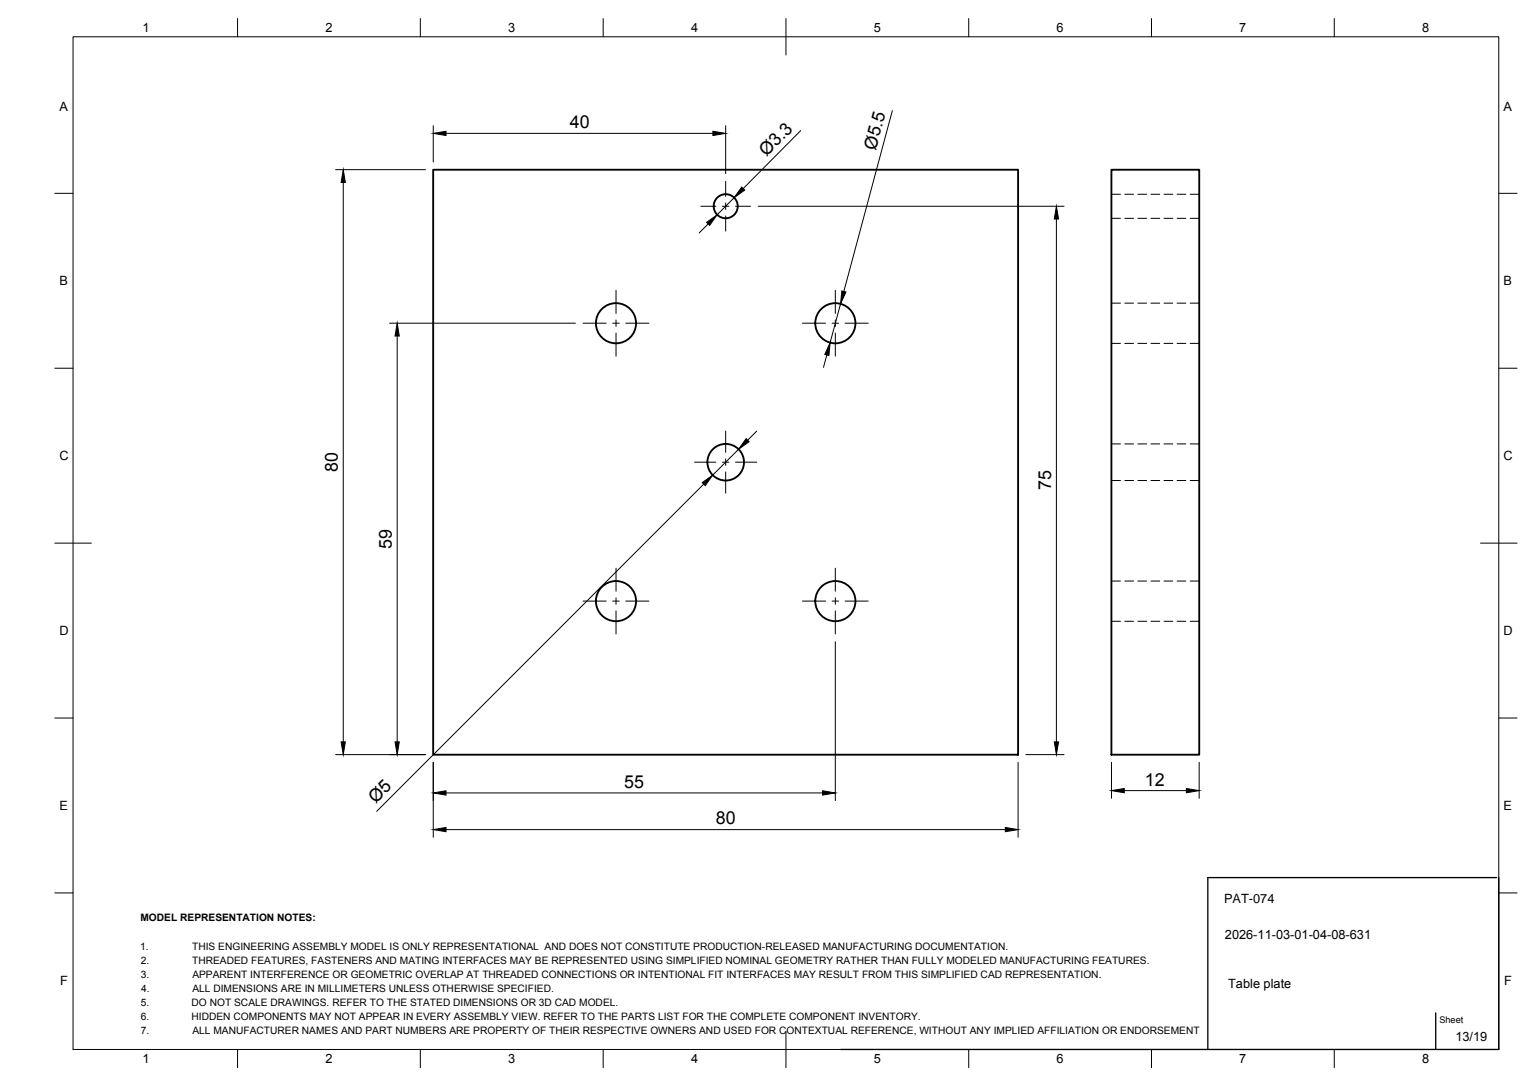
ISO-10303-21;
HEADER;
/* Generated by software containing ST-Developer
 * from STEP Tools, Inc. (www.steptools.com) 
 */

FILE_DESCRIPTION(
/* description */ ('Manual rail carriage with stops'),
/* implementation_level */ '2;1');

FILE_NAME(
/* name */ 'Table plate.step',
/* time_stamp */ '2026-10-27T18:54:27-07:00',
/* author */ (''),
/* organization */ (''),
/* preprocessor_version */ 'ST-DEVELOPER v20.2',
/* originating_system */ 'Autodesk Translation Framework v15.17.0.0',
/* authorisation */ '');

FILE_SCHEMA (('AUTOMOTIVE_DESIGN { 1 0 10303 214 3 1 1 }'));
ENDSEC;

DATA;
#10=MECHANICAL_DESIGN_GEOMETRIC_PRESENTATION_REPRESENTATION('',(#285),#8499);
#249=SHAPE_REPRESENTATION_RELATIONSHIP('SRR','None',#8614,#267);
#267=ADVANCED_BREP_SHAPE_REPRESENTATION('',(#301),#8493);
#285=STYLED_ITEM('',(#8781),#301);
#301=MANIFOLD_SOLID_BREP('Body1',#4955);
#360=FACE_BOUND('',#1114,.T.);
#361=FACE_BOUND('',#1115,.T.);
#362=FACE_BOUND('',#1116,.T.);
#363=FACE_BOUND('',#1117,.T.);
#364=FACE_BOUND('',#1118,.T.);
#365=FACE_BOUND('',#1119,.T.);
#366=FACE_BOUND('',#1121,.T.);
#367=FACE_BOUND('',#1122,.T.);
#368=FACE_BOUND('',#1123,.T.);
#369=FACE_BOUND('',#1124,.T.);
#370=FACE_BOUND('',#1125,.T.);
#371=FACE_BOUND('',#1126,.T.);
#543=PLANE('',#5497);
#544=PLANE('',#5498);
#545=PLANE('',#5499);
#546=PLANE('',#5500);
#547=PLANE('',#5501);
#548=PLANE('',#5502);
#783=FACE_OUTER_BOUND('',#1103,.T.);
#784=FACE_OUTER_BOUND('',#1104,.T.);
#785=FACE_OUTER_BOUND('',#1105,.T.);
#786=FACE_OUTER_BOUND('',#1106,.T.);
#787=FACE_OUTER_BOUND('',#1107,.T.);
#788=FACE_OUTER_BOUND('',#1108,.T.);
#789=FACE_OUTER_BOUND('',#1109,.T.);
#790=FACE_OUTER_BOUND('',#1110,.T.);
#791=FACE_OUTER_BOUND('',#1111,.T.);
#792=FACE_OUTER_BOUND('',#1112,.T.);
#793=FACE_OUTER_BOUND('',#1113,.T.);
#794=FACE_OUTER_BOUND('',#1120,.T.);
#1103=EDGE_LOOP('',(#4396,#4397,#4398,#4399));
#1104=EDGE_LOOP('',(#4400,#4401,#4402,#4403));
#1105=EDGE_LOOP('',(#4404,#4405,#4406,#4407));
#1106=EDGE_LOOP('',(#4408,#4409,#4410,#4411));
#1107=EDGE_LOOP('',(#4412,#4413,#4414,#4415));
#1108=EDGE_LOOP('',(#4416,#4417,#4418,#4419));
#1109=EDGE_LOOP('',(#4420,#4421,#4422,#4423));
#1110=EDGE_LOOP('',(#4424,#4425,#4426,#4427));
#1111=EDGE_LOOP('',(#4428,#4429,#4430,#4431));
#1112=EDGE_LOOP('',(#4432,#4433,#4434,#4435));
#1113=EDGE_LOOP('',(#4436,#4437,#4438,#4439));
#1114=EDGE_LOOP('',(#4440));
#1115=EDGE_LOOP('',(#4441));
#1116=EDGE_LOOP('',(#4442));
#1117=EDGE_LOOP('',(#4443));
#1118=EDGE_LOOP('',(#4444));
#1119=EDGE_LOOP('',(#4445));
#1120=EDGE_LOOP('',(#4446,#4447,#4448,#4449));
#1121=EDGE_LOOP('',(#4450));
#1122=EDGE_LOOP('',(#4451));
#1123=EDGE_LOOP('',(#4452));
#1124=EDGE_LOOP('',(#4453));
#1125=EDGE_LOOP('',(#4454));
#1126=EDGE_LOOP('',(#4455));
#1609=LINE('',#8160,#2109);
#1610=LINE('',#8166,#2110);
#1611=LINE('',#8172,#2111);
#1612=LINE('',#8178,#2112);
#1613=LINE('',#8184,#2113);
#1614=LINE('',#8190,#2114);
#1615=LINE('',#8195,#2115);
#1616=LINE('',#8197,#2116);
#1617=LINE('',#8199,#2117);
#1618=LINE('',#8200,#2118);
#1619=LINE('',#8203,#2119);
#1620=LINE('',#8205,#2120);
#1621=LINE('',#8206,#2121);
#1622=LINE('',#8209,#2122);
#1623=LINE('',#8211,#2123);
#1624=LINE('',#8212,#2124);
#1625=LINE('',#8214,#2125);
#1626=LINE('',#8215,#2126);
#2109=VECTOR('',#6696,0.164999999999999);
#2110=VECTOR('',#6703,0.25);
#2111=VECTOR('',#6710,0.275);
#2112=VECTOR('',#6717,0.275);
#2113=VECTOR('',#6724,0.275);
#2114=VECTOR('',#6731,0.275);
#2115=VECTOR('',#6736,1.);
#2116=VECTOR('',#6737,1.);
#2117=VECTOR('',#6738,1.);
#2118=VECTOR('',#6739,1.);
#2119=VECTOR('',#6742,1.);
#2120=VECTOR('',#6743,1.);
#2121=VECTOR('',#6744,1.);
#2122=VECTOR('',#6747,1.);
#2123=VECTOR('',#6748,1.);
#2124=VECTOR('',#6749,1.);
#2125=VECTOR('',#6752,1.);
#2126=VECTOR('',#6753,1.);
#2271=CIRCLE('',#5480,0.164999999999999);
#2272=CIRCLE('',#5481,0.164999999999999);
#2273=CIRCLE('',#5483,0.25);
#2274=CIRCLE('',#5484,0.25);
#2275=CIRCLE('',#5486,0.275);
#2276=CIRCLE('',#5487,0.275);
#2277=CIRCLE('',#5489,0.275);
#2278=CIRCLE('',#5490,0.275);
#2279=CIRCLE('',#5492,0.275);
#2280=CIRCLE('',#5493,0.275);
#2281=CIRCLE('',#5495,0.275);
#2282=CIRCLE('',#5496,0.275);
#2655=VERTEX_POINT('',#8157);
#2656=VERTEX_POINT('',#8159);
#2657=VERTEX_POINT('',#8163);
#2658=VERTEX_POINT('',#8165);
#2659=VERTEX_POINT('',#8169);
#2660=VERTEX_POINT('',#8171);
#2661=VERTEX_POINT('',#8175);
#2662=VERTEX_POINT('',#8177);
#2663=VERTEX_POINT('',#8181);
#2664=VERTEX_POINT('',#8183);
#2665=VERTEX_POINT('',#8187);
#2666=VERTEX_POINT('',#8189);
#2667=VERTEX_POINT('',#8193);
#2668=VERTEX_POINT('',#8194);
#2669=VERTEX_POINT('',#8196);
#2670=VERTEX_POINT('',#8198);
#2671=VERTEX_POINT('',#8202);
#2672=VERTEX_POINT('',#8204);
#2673=VERTEX_POINT('',#8208);
#2674=VERTEX_POINT('',#8210);
#3246=EDGE_CURVE('',#2655,#2655,#2271,.T.);
#3247=EDGE_CURVE('',#2655,#2656,#1609,.T.);
#3248=EDGE_CURVE('',#2656,#2656,#2272,.T.);
#3249=EDGE_CURVE('',#2657,#2657,#2273,.T.);
#3250=EDGE_CURVE('',#2657,#2658,#1610,.T.);
#3251=EDGE_CURVE('',#2658,#2658,#2274,.T.);
#3252=EDGE_CURVE('',#2659,#2659,#2275,.T.);
#3253=EDGE_CURVE('',#2659,#2660,#1611,.T.);
#3254=EDGE_CURVE('',#2660,#2660,#2276,.T.);
#3255=EDGE_CURVE('',#2661,#2661,#2277,.T.);
#3256=EDGE_CURVE('',#2661,#2662,#1612,.T.);
#3257=EDGE_CURVE('',#2662,#2662,#2278,.T.);
#3258=EDGE_CURVE('',#2663,#2663,#2279,.T.);
#3259=EDGE_CURVE('',#2663,#2664,#1613,.T.);
#3260=EDGE_CURVE('',#2664,#2664,#2280,.T.);
#3261=EDGE_CURVE('',#2665,#2665,#2281,.T.);
#3262=EDGE_CURVE('',#2665,#2666,#1614,.T.);
#3263=EDGE_CURVE('',#2666,#2666,#2282,.T.);
#3264=EDGE_CURVE('',#2667,#2668,#1615,.T.);
#3265=EDGE_CURVE('',#2668,#2669,#1616,.T.);
#3266=EDGE_CURVE('',#2670,#2669,#1617,.T.);
#3267=EDGE_CURVE('',#2667,#2670,#1618,.T.);
#3268=EDGE_CURVE('',#2671,#2667,#1619,.T.);
#3269=EDGE_CURVE('',#2672,#2670,#1620,.T.);
#3270=EDGE_CURVE('',#2671,#2672,#1621,.T.);
#3271=EDGE_CURVE('',#2673,#2671,#1622,.T.);
#3272=EDGE_CURVE('',#2674,#2672,#1623,.T.);
#3273=EDGE_CURVE('',#2673,#2674,#1624,.T.);
#3274=EDGE_CURVE('',#2668,#2673,#1625,.T.);
#3275=EDGE_CURVE('',#2669,#2674,#1626,.T.);
#4396=ORIENTED_EDGE('',*,*,#3246,.F.);
#4397=ORIENTED_EDGE('',*,*,#3247,.T.);
#4398=ORIENTED_EDGE('',*,*,#3248,.F.);
#4399=ORIENTED_EDGE('',*,*,#3247,.F.);
#4400=ORIENTED_EDGE('',*,*,#3249,.F.);
#4401=ORIENTED_EDGE('',*,*,#3250,.T.);
#4402=ORIENTED_EDGE('',*,*,#3251,.F.);
#4403=ORIENTED_EDGE('',*,*,#3250,.F.);
#4404=ORIENTED_EDGE('',*,*,#3252,.F.);
#4405=ORIENTED_EDGE('',*,*,#3253,.T.);
#4406=ORIENTED_EDGE('',*,*,#3254,.F.);
#4407=ORIENTED_EDGE('',*,*,#3253,.F.);
#4408=ORIENTED_EDGE('',*,*,#3255,.F.);
#4409=ORIENTED_EDGE('',*,*,#3256,.T.);
#4410=ORIENTED_EDGE('',*,*,#3257,.F.);
#4411=ORIENTED_EDGE('',*,*,#3256,.F.);
#4412=ORIENTED_EDGE('',*,*,#3258,.F.);
#4413=ORIENTED_EDGE('',*,*,#3259,.T.);
#4414=ORIENTED_EDGE('',*,*,#3260,.F.);
#4415=ORIENTED_EDGE('',*,*,#3259,.F.);
#4416=ORIENTED_EDGE('',*,*,#3261,.F.);
#4417=ORIENTED_EDGE('',*,*,#3262,.T.);
#4418=ORIENTED_EDGE('',*,*,#3263,.F.);
#4419=ORIENTED_EDGE('',*,*,#3262,.F.);
#4420=ORIENTED_EDGE('',*,*,#3264,.T.);
#4421=ORIENTED_EDGE('',*,*,#3265,.T.);
#4422=ORIENTED_EDGE('',*,*,#3266,.F.);
#4423=ORIENTED_EDGE('',*,*,#3267,.F.);
#4424=ORIENTED_EDGE('',*,*,#3268,.T.);
#4425=ORIENTED_EDGE('',*,*,#3267,.T.);
#4426=ORIENTED_EDGE('',*,*,#3269,.F.);
#4427=ORIENTED_EDGE('',*,*,#3270,.F.);
#4428=ORIENTED_EDGE('',*,*,#3271,.T.);
#4429=ORIENTED_EDGE('',*,*,#3270,.T.);
#4430=ORIENTED_EDGE('',*,*,#3272,.F.);
#4431=ORIENTED_EDGE('',*,*,#3273,.F.);
#4432=ORIENTED_EDGE('',*,*,#3274,.T.);
#4433=ORIENTED_EDGE('',*,*,#3273,.T.);
#4434=ORIENTED_EDGE('',*,*,#3275,.F.);
#4435=ORIENTED_EDGE('',*,*,#3265,.F.);
#4436=ORIENTED_EDGE('',*,*,#3275,.T.);
#4437=ORIENTED_EDGE('',*,*,#3272,.T.);
#4438=ORIENTED_EDGE('',*,*,#3269,.T.);
#4439=ORIENTED_EDGE('',*,*,#3266,.T.);
#4440=ORIENTED_EDGE('',*,*,#3248,.T.);
#4441=ORIENTED_EDGE('',*,*,#3251,.T.);
#4442=ORIENTED_EDGE('',*,*,#3254,.T.);
#4443=ORIENTED_EDGE('',*,*,#3257,.T.);
#4444=ORIENTED_EDGE('',*,*,#3260,.T.);
#4445=ORIENTED_EDGE('',*,*,#3263,.T.);
#4446=ORIENTED_EDGE('',*,*,#3274,.F.);
#4447=ORIENTED_EDGE('',*,*,#3264,.F.);
#4448=ORIENTED_EDGE('',*,*,#3268,.F.);
#4449=ORIENTED_EDGE('',*,*,#3271,.F.);
#4450=ORIENTED_EDGE('',*,*,#3246,.T.);
#4451=ORIENTED_EDGE('',*,*,#3249,.T.);
#4452=ORIENTED_EDGE('',*,*,#3252,.T.);
#4453=ORIENTED_EDGE('',*,*,#3255,.T.);
#4454=ORIENTED_EDGE('',*,*,#3258,.T.);
#4455=ORIENTED_EDGE('',*,*,#3261,.T.);
#4660=CYLINDRICAL_SURFACE('',#5479,0.164999999999999);
#4661=CYLINDRICAL_SURFACE('',#5482,0.25);
#4662=CYLINDRICAL_SURFACE('',#5485,0.275);
#4663=CYLINDRICAL_SURFACE('',#5488,0.275);
#4664=CYLINDRICAL_SURFACE('',#5491,0.275);
#4665=CYLINDRICAL_SURFACE('',#5494,0.275);
#4882=ADVANCED_FACE('',(#783),#4660,.F.);
#4883=ADVANCED_FACE('',(#784),#4661,.F.);
#4884=ADVANCED_FACE('',(#785),#4662,.F.);
#4885=ADVANCED_FACE('',(#786),#4663,.F.);
#4886=ADVANCED_FACE('',(#787),#4664,.F.);
#4887=ADVANCED_FACE('',(#788),#4665,.F.);
#4888=ADVANCED_FACE('',(#789),#543,.T.);
#4889=ADVANCED_FACE('',(#790),#544,.T.);
#4890=ADVANCED_FACE('',(#791),#545,.T.);
#4891=ADVANCED_FACE('',(#792),#546,.T.);
#4892=ADVANCED_FACE('',(#793,#360,#361,#362,#363,#364,#365),#547,.T.);
#4893=ADVANCED_FACE('',(#794,#366,#367,#368,#369,#370,#371),#548,.F.);
#4955=CLOSED_SHELL('',(#4882,#4883,#4884,#4885,#4886,#4887,#4888,#4889,
#4890,#4891,#4892,#4893));
#5478=AXIS2_PLACEMENT_3D('',#8155,#6690,#6691);
#5479=AXIS2_PLACEMENT_3D('',#8156,#6692,#6693);
#5480=AXIS2_PLACEMENT_3D('',#8158,#6694,#6695);
#5481=AXIS2_PLACEMENT_3D('',#8161,#6697,#6698);
#5482=AXIS2_PLACEMENT_3D('',#8162,#6699,#6700);
#5483=AXIS2_PLACEMENT_3D('',#8164,#6701,#6702);
#5484=AXIS2_PLACEMENT_3D('',#8167,#6704,#6705);
#5485=AXIS2_PLACEMENT_3D('',#8168,#6706,#6707);
#5486=AXIS2_PLACEMENT_3D('',#8170,#6708,#6709);
#5487=AXIS2_PLACEMENT_3D('',#8173,#6711,#6712);
#5488=AXIS2_PLACEMENT_3D('',#8174,#6713,#6714);
#5489=AXIS2_PLACEMENT_3D('',#8176,#6715,#6716);
#5490=AXIS2_PLACEMENT_3D('',#8179,#6718,#6719);
#5491=AXIS2_PLACEMENT_3D('',#8180,#6720,#6721);
#5492=AXIS2_PLACEMENT_3D('',#8182,#6722,#6723);
#5493=AXIS2_PLACEMENT_3D('',#8185,#6725,#6726);
#5494=AXIS2_PLACEMENT_3D('',#8186,#6727,#6728);
#5495=AXIS2_PLACEMENT_3D('',#8188,#6729,#6730);
#5496=AXIS2_PLACEMENT_3D('',#8191,#6732,#6733);
#5497=AXIS2_PLACEMENT_3D('',#8192,#6734,#6735);
#5498=AXIS2_PLACEMENT_3D('',#8201,#6740,#6741);
#5499=AXIS2_PLACEMENT_3D('',#8207,#6745,#6746);
#5500=AXIS2_PLACEMENT_3D('',#8213,#6750,#6751);
#5501=AXIS2_PLACEMENT_3D('',#8216,#6754,#6755);
#5502=AXIS2_PLACEMENT_3D('',#8217,#6756,#6757);
#6690=DIRECTION('axis',(0.,0.,1.));
#6691=DIRECTION('refdir',(1.,0.,0.));
#6692=DIRECTION('center_axis',(0.,0.,1.));
#6693=DIRECTION('ref_axis',(1.,0.,0.));
#6694=DIRECTION('center_axis',(0.,0.,1.));
#6695=DIRECTION('ref_axis',(1.,0.,0.));
#6696=DIRECTION('',(0.,0.,1.));
#6697=DIRECTION('center_axis',(0.,0.,-1.));
#6698=DIRECTION('ref_axis',(1.,0.,0.));
#6699=DIRECTION('center_axis',(0.,0.,1.));
#6700=DIRECTION('ref_axis',(1.,0.,0.));
#6701=DIRECTION('center_axis',(0.,0.,1.));
#6702=DIRECTION('ref_axis',(1.,0.,0.));
#6703=DIRECTION('',(0.,0.,1.));
#6704=DIRECTION('center_axis',(0.,0.,-1.));
#6705=DIRECTION('ref_axis',(1.,0.,0.));
#6706=DIRECTION('center_axis',(0.,0.,1.));
#6707=DIRECTION('ref_axis',(1.,0.,0.));
#6708=DIRECTION('center_axis',(0.,0.,1.));
#6709=DIRECTION('ref_axis',(1.,0.,0.));
#6710=DIRECTION('',(0.,0.,1.));
#6711=DIRECTION('center_axis',(0.,0.,-1.));
#6712=DIRECTION('ref_axis',(1.,0.,0.));
#6713=DIRECTION('center_axis',(0.,0.,1.));
#6714=DIRECTION('ref_axis',(1.,0.,0.));
#6715=DIRECTION('center_axis',(0.,0.,1.));
#6716=DIRECTION('ref_axis',(1.,0.,0.));
#6717=DIRECTION('',(0.,0.,1.));
#6718=DIRECTION('center_axis',(0.,0.,-1.));
#6719=DIRECTION('ref_axis',(1.,0.,0.));
#6720=DIRECTION('center_axis',(0.,0.,1.));
#6721=DIRECTION('ref_axis',(1.,0.,0.));
#6722=DIRECTION('center_axis',(0.,0.,1.));
#6723=DIRECTION('ref_axis',(1.,0.,0.));
#6724=DIRECTION('',(0.,0.,1.));
#6725=DIRECTION('center_axis',(0.,0.,-1.));
#6726=DIRECTION('ref_axis',(1.,0.,0.));
#6727=DIRECTION('center_axis',(0.,0.,1.));
#6728=DIRECTION('ref_axis',(1.,0.,0.));
#6729=DIRECTION('center_axis',(0.,0.,1.));
#6730=DIRECTION('ref_axis',(1.,0.,0.));
#6731=DIRECTION('',(0.,0.,1.));
#6732=DIRECTION('center_axis',(0.,0.,-1.));
#6733=DIRECTION('ref_axis',(1.,0.,0.));
#6734=DIRECTION('center_axis',(0.,1.,0.));
#6735=DIRECTION('ref_axis',(-1.,0.,0.));
#6736=DIRECTION('',(-1.,0.,0.));
#6737=DIRECTION('',(0.,0.,1.));
#6738=DIRECTION('',(-1.,0.,0.));
#6739=DIRECTION('',(0.,0.,1.));
#6740=DIRECTION('center_axis',(1.,0.,0.));
#6741=DIRECTION('ref_axis',(0.,1.,0.));
#6742=DIRECTION('',(0.,1.,0.));
#6743=DIRECTION('',(0.,1.,0.));
#6744=DIRECTION('',(0.,0.,1.));
#6745=DIRECTION('center_axis',(0.,-1.,0.));
#6746=DIRECTION('ref_axis',(1.,0.,0.));
#6747=DIRECTION('',(1.,0.,0.));
#6748=DIRECTION('',(1.,0.,0.));
#6749=DIRECTION('',(0.,0.,1.));
#6750=DIRECTION('center_axis',(-1.,0.,0.));
#6751=DIRECTION('ref_axis',(0.,-1.,0.));
#6752=DIRECTION('',(0.,-1.,0.));
#6753=DIRECTION('',(0.,-1.,0.));
#6754=DIRECTION('center_axis',(0.,0.,1.));
#6755=DIRECTION('ref_axis',(1.,0.,0.));
#6756=DIRECTION('center_axis',(0.,0.,1.));
#6757=DIRECTION('ref_axis',(1.,0.,0.));
#8155=CARTESIAN_POINT('',(0.,0.,0.));
#8156=CARTESIAN_POINT('Origin',(11.,3.5,5.1));
#8157=CARTESIAN_POINT('',(10.835,3.5,5.2));
#8158=CARTESIAN_POINT('Origin',(11.,3.5,5.2));
#8159=CARTESIAN_POINT('',(10.835,3.5,6.4));
#8160=CARTESIAN_POINT('',(10.835,3.5,5.1));
#8161=CARTESIAN_POINT('Origin',(11.,3.5,6.4));
#8162=CARTESIAN_POINT('Origin',(11.,0.,5.1));
#8163=CARTESIAN_POINT('',(10.75,-3.06161699786838E-17,5.2));
#8164=CARTESIAN_POINT('Origin',(11.,0.,5.2));
#8165=CARTESIAN_POINT('',(10.75,3.06161699786838E-17,6.4));
#8166=CARTESIAN_POINT('',(10.75,-3.06161699786838E-17,5.1));
#8167=CARTESIAN_POINT('Origin',(11.,0.,6.4));
#8168=CARTESIAN_POINT('Origin',(12.5,-1.9,5.1));
#8169=CARTESIAN_POINT('',(12.225,-1.9,5.2));
#8170=CARTESIAN_POINT('Origin',(12.5,-1.9,5.2));
#8171=CARTESIAN_POINT('',(12.225,-1.9,6.4));
#8172=CARTESIAN_POINT('',(12.225,-1.9,5.1));
#8173=CARTESIAN_POINT('Origin',(12.5,-1.9,6.4));
#8174=CARTESIAN_POINT('Origin',(9.5,1.9,5.1));
#8175=CARTESIAN_POINT('',(9.225,1.9,5.2));
#8176=CARTESIAN_POINT('Origin',(9.5,1.9,5.2));
#8177=CARTESIAN_POINT('',(9.225,1.9,6.4));
#8178=CARTESIAN_POINT('',(9.225,1.9,5.1));
#8179=CARTESIAN_POINT('Origin',(9.5,1.9,6.4));
#8180=CARTESIAN_POINT('Origin',(9.5,-1.9,5.1));
#8181=CARTESIAN_POINT('',(9.225,-1.9,5.2));
#8182=CARTESIAN_POINT('Origin',(9.5,-1.9,5.2));
#8183=CARTESIAN_POINT('',(9.225,-1.9,6.4));
#8184=CARTESIAN_POINT('',(9.225,-1.9,5.1));
#8185=CARTESIAN_POINT('Origin',(9.5,-1.9,6.4));
#8186=CARTESIAN_POINT('Origin',(12.5,1.9,5.1));
#8187=CARTESIAN_POINT('',(12.225,1.9,5.2));
#8188=CARTESIAN_POINT('Origin',(12.5,1.9,5.2));
#8189=CARTESIAN_POINT('',(12.225,1.9,6.4));
#8190=CARTESIAN_POINT('',(12.225,1.9,5.1));
#8191=CARTESIAN_POINT('Origin',(12.5,1.9,6.4));
#8192=CARTESIAN_POINT('Origin',(15.,4.,5.2));
#8193=CARTESIAN_POINT('',(15.,4.,5.2));
#8194=CARTESIAN_POINT('',(7.,4.,5.2));
#8195=CARTESIAN_POINT('',(15.,4.,5.2));
#8196=CARTESIAN_POINT('',(7.,4.,6.4));
#8197=CARTESIAN_POINT('',(7.,4.,5.2));
#8198=CARTESIAN_POINT('',(15.,4.,6.4));
#8199=CARTESIAN_POINT('',(15.,4.,6.4));
#8200=CARTESIAN_POINT('',(15.,4.,5.2));
#8201=CARTESIAN_POINT('Origin',(15.,-4.,5.2));
#8202=CARTESIAN_POINT('',(15.,-4.,5.2));
#8203=CARTESIAN_POINT('',(15.,-4.,5.2));
#8204=CARTESIAN_POINT('',(15.,-4.,6.4));
#8205=CARTESIAN_POINT('',(15.,-4.,6.4));
#8206=CARTESIAN_POINT('',(15.,-4.,5.2));
#8207=CARTESIAN_POINT('Origin',(7.,-4.,5.2));
#8208=CARTESIAN_POINT('',(7.,-4.,5.2));
#8209=CARTESIAN_POINT('',(7.,-4.,5.2));
#8210=CARTESIAN_POINT('',(7.,-4.,6.4));
#8211=CARTESIAN_POINT('',(7.,-4.,6.4));
#8212=CARTESIAN_POINT('',(7.,-4.,5.2));
#8213=CARTESIAN_POINT('Origin',(7.,4.,5.2));
#8214=CARTESIAN_POINT('',(7.,4.,5.2));
#8215=CARTESIAN_POINT('',(7.,4.,6.4));
#8216=CARTESIAN_POINT('Origin',(11.,0.,6.4));
#8217=CARTESIAN_POINT('Origin',(11.,0.,5.2));
#8470=UNCERTAINTY_MEASURE_WITH_UNIT(LENGTH_MEASURE(0.001),#8500,
'DISTANCE_ACCURACY_VALUE',
'Maximum model space distance between geometric entities at asserted c
onnectivities');
#8476=UNCERTAINTY_MEASURE_WITH_UNIT(LENGTH_MEASURE(0.001),#8500,
'DISTANCE_ACCURACY_VALUE',
'Maximum model space distance between geometric entities at asserted c
onnectivities');
#8493=(
GEOMETRIC_REPRESENTATION_CONTEXT(3)
GLOBAL_UNCERTAINTY_ASSIGNED_CONTEXT((#8470))
GLOBAL_UNIT_ASSIGNED_CONTEXT((#8500,#8502,#8503))
REPRESENTATION_CONTEXT('','3D')
);
#8499=(
GEOMETRIC_REPRESENTATION_CONTEXT(3)
GLOBAL_UNCERTAINTY_ASSIGNED_CONTEXT((#8476))
GLOBAL_UNIT_ASSIGNED_CONTEXT((#8500,#8502,#8503))
REPRESENTATION_CONTEXT('','3D')
);
#8500=(
LENGTH_UNIT()
NAMED_UNIT(*)
SI_UNIT(.CENTI.,.METRE.)
);
#8502=(
NAMED_UNIT(*)
PLANE_ANGLE_UNIT()
SI_UNIT($,.RADIAN.)
);
#8503=(
NAMED_UNIT(*)
SI_UNIT($,.STERADIAN.)
SOLID_ANGLE_UNIT()
);
#8520=SHAPE_DEFINITION_REPRESENTATION(#8545,#8614);
#8545=PRODUCT_DEFINITION_SHAPE('',$,#8637);
#8614=SHAPE_REPRESENTATION('',(#5478),#8493);
#8620=PRODUCT_DEFINITION_CONTEXT('part definition',#8688,'design');
#8637=PRODUCT_DEFINITION('Table plate','Table plate',#8659,#8620);
#8659=PRODUCT_DEFINITION_FORMATION('',$,#8706);
#8688=APPLICATION_CONTEXT(
'Core Data for Automotive Mechanical Design Process');
#8689=PRODUCT_CONTEXT('part definition',#8688,'mechanical');
#8706=PRODUCT('Table plate','Table plate','Table plate',(#8689));
#8775=COLOUR_RGB('Sky Blue',0.24,0.69,0.87);
#8776=FILL_AREA_STYLE_COLOUR('',#8775);
#8777=FILL_AREA_STYLE('',(#8776));
#8778=SURFACE_STYLE_FILL_AREA(#8777);
#8779=SURFACE_SIDE_STYLE('',(#8778));
#8780=SURFACE_STYLE_USAGE(.BOTH.,#8779);
#8781=PRESENTATION_STYLE_ASSIGNMENT((#8780));
ENDSEC;
END-ISO-10303-21;
